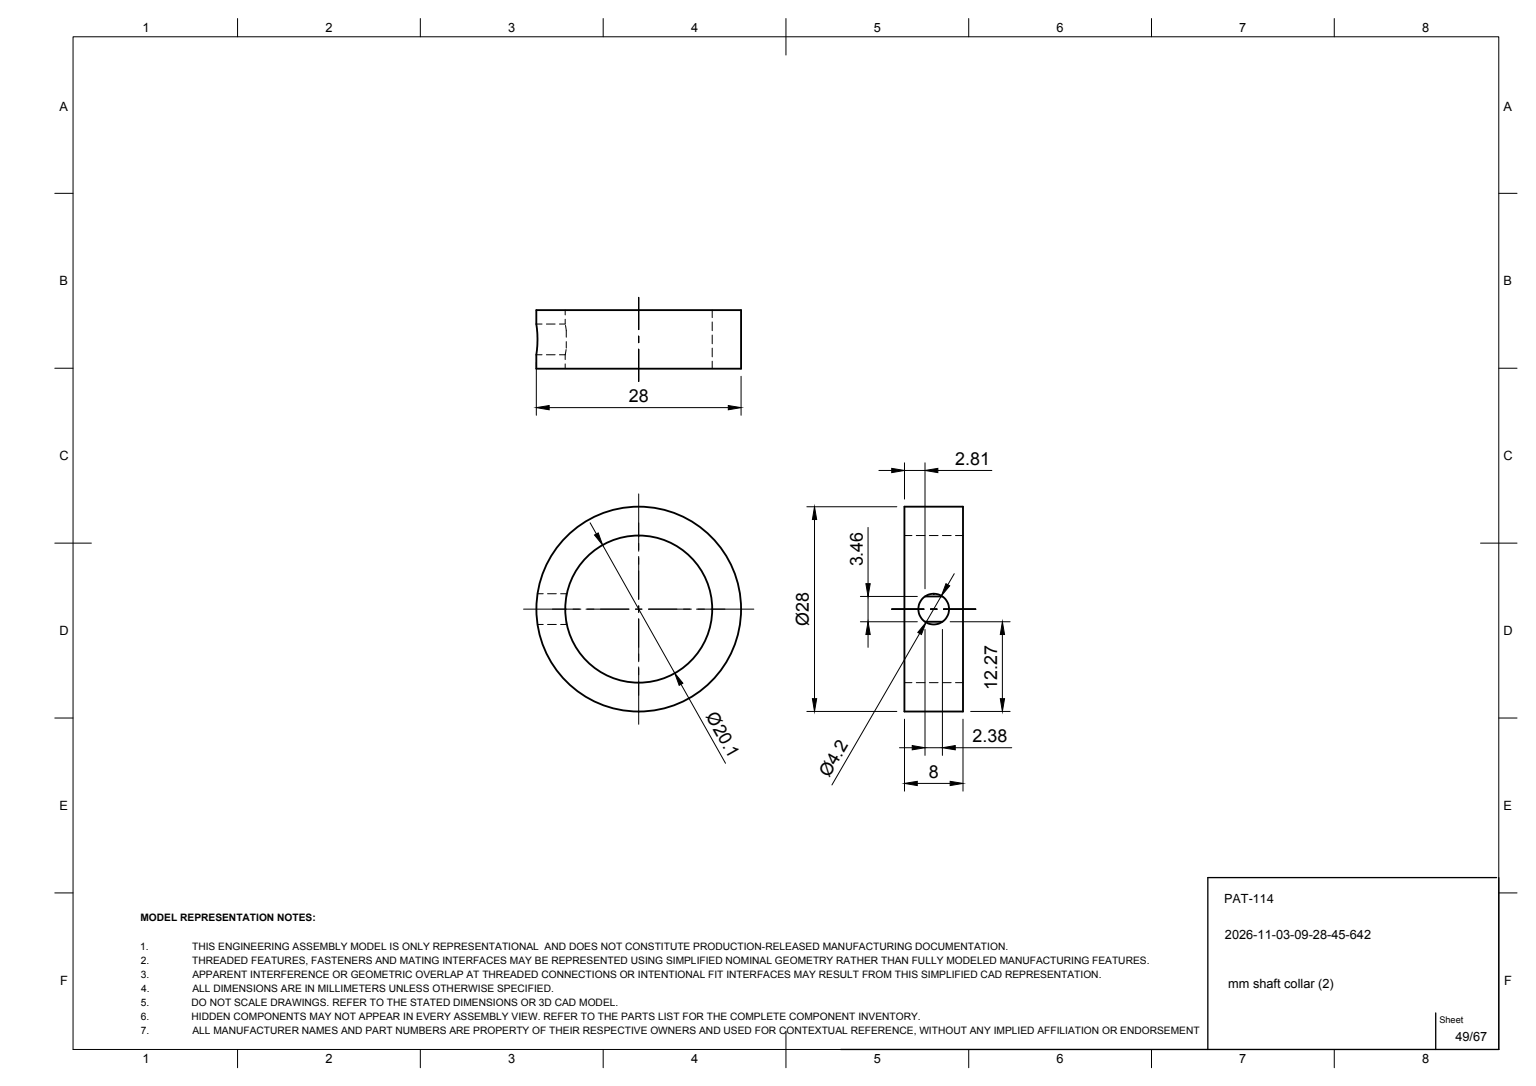
ISO-10303-21;
HEADER;
/* Generated by software containing ST-Developer
 * from STEP Tools, Inc. (www.steptools.com) 
 */

FILE_DESCRIPTION(
/* description */ ('Two-stage gear reducer in split housing'),
/* implementation_level */ '2;1');

FILE_NAME(
/* name */ 'mm shaft collar (2).step',
/* time_stamp */ '2026-10-28T03:22:31-07:00',
/* author */ (''),
/* organization */ (''),
/* preprocessor_version */ 'ST-DEVELOPER v20.2',
/* originating_system */ 'Autodesk Translation Framework v15.17.0.0',
/* authorisation */ '');

FILE_SCHEMA (('AUTOMOTIVE_DESIGN { 1 0 10303 214 3 1 1 }'));
ENDSEC;

DATA;
#10=MECHANICAL_DESIGN_GEOMETRIC_PRESENTATION_REPRESENTATION('',(#1287),#73366);
#971=B_SPLINE_CURVE_WITH_KNOTS('',3,(#37404,#37405,#37406,#37407,#37408,
#37409,#37410,#37411,#37412,#37413,#37414,#37415,#37416,#37417),
 .UNSPECIFIED.,.F.,.F.,(4,2,2,2,2,2,4),(0.756005737987032,0.793568827564648,
0.872922520054202,0.952276212543757,1.03162990503331,1.11098359752287,1.14854668710048),
 .UNSPECIFIED.);
#972=B_SPLINE_CURVE_WITH_KNOTS('',3,(#37423,#37424,#37425,#37426,#37427,
#37428,#37429,#37430,#37431,#37432,#37433,#37434,#37435,#37436,#37437,#37438,
#37439,#37440),.UNSPECIFIED.,.F.,.F.,(4,2,2,2,2,2,2,2,4),(0.,0.0792334805614376,
0.158466961122875,0.237699060165218,0.31693115920756,0.396163258249903,
0.475395357292245,0.554628837853683,0.633862318415121),.UNSPECIFIED.);
#973=B_SPLINE_CURVE_WITH_KNOTS('',3,(#37441,#37442,#37443,#37444,#37445,
#37446,#37447,#37448,#37449,#37450,#37451,#37452,#37453,#37454,#37455,#37456,
#37457,#37458),.UNSPECIFIED.,.F.,.F.,(4,2,2,2,2,2,2,2,4),(0.633862318415121,
0.713095798976558,0.792329279537995,0.871561378580338,0.950793477622681,
1.03002557666502,1.10925767570737,1.1884911562688,1.26772463683024),
 .UNSPECIFIED.);
#974=B_SPLINE_CURVE_WITH_KNOTS('',3,(#37461,#37462,#37463,#37464,#37465,
#37466,#37467,#37468,#37469,#37470,#37471,#37472,#37473,#37474),
 .UNSPECIFIED.,.F.,.F.,(4,2,2,2,2,2,4),(0.121154929624526,0.158718019202143,
0.238071711691697,0.317425404181252,0.396779096670807,0.476132789160362,
0.51369587873798),.UNSPECIFIED.);
#1160=SHAPE_REPRESENTATION_RELATIONSHIP('SRR','None',#73651,#1216);
#1216=ADVANCED_BREP_SHAPE_REPRESENTATION('',(#1356),#73347);
#1287=STYLED_ITEM('',(#73988),#1356);
#1356=MANIFOLD_SOLID_BREP('Body1',#16177);
#1560=FACE_BOUND('',#3668,.T.);
#1561=FACE_BOUND('',#3670,.T.);
#1562=FACE_BOUND('',#3672,.T.);
#1563=FACE_BOUND('',#3674,.T.);
#1870=PLANE('',#17970);
#1871=PLANE('',#17975);
#1872=PLANE('',#17982);
#1873=PLANE('',#17983);
#2565=FACE_OUTER_BOUND('',#3664,.T.);
#2566=FACE_OUTER_BOUND('',#3665,.T.);
#2567=FACE_OUTER_BOUND('',#3666,.T.);
#2568=FACE_OUTER_BOUND('',#3667,.T.);
#2569=FACE_OUTER_BOUND('',#3669,.T.);
#2570=FACE_OUTER_BOUND('',#3671,.T.);
#2571=FACE_OUTER_BOUND('',#3673,.T.);
#3664=EDGE_LOOP('',(#13043,#13044));
#3665=EDGE_LOOP('',(#13045,#13046,#13047,#13048,#13049,#13050,#13051,#13052,
#13053));
#3666=EDGE_LOOP('',(#13054,#13055,#13056));
#3667=EDGE_LOOP('',(#13057,#13058,#13059,#13060));
#3668=EDGE_LOOP('',(#13061,#13062,#13063,#13064));
#3669=EDGE_LOOP('',(#13065,#13066,#13067,#13068));
#3670=EDGE_LOOP('',(#13069,#13070));
#3671=EDGE_LOOP('',(#13071));
#3672=EDGE_LOOP('',(#13072));
#3673=EDGE_LOOP('',(#13073));
#3674=EDGE_LOOP('',(#13074));
#4684=LINE('',#37400,#5708);
#4685=LINE('',#37421,#5709);
#4686=LINE('',#37476,#5710);
#4687=LINE('',#37481,#5711);
#4688=LINE('',#37487,#5712);
#5708=VECTOR('',#21404,1.);
#5709=VECTOR('',#21411,0.21);
#5710=VECTOR('',#21416,1.);
#5711=VECTOR('',#21421,1.005);
#5712=VECTOR('',#21428,1.4);
#6624=CIRCLE('',#17971,0.21);
#6625=CIRCLE('',#17973,0.21);
#6626=CIRCLE('',#17974,0.21);
#6627=CIRCLE('',#17977,1.005);
#6628=CIRCLE('',#17978,1.005);
#6629=CIRCLE('',#17980,1.4);
#6630=CIRCLE('',#17981,1.4);
#7685=VERTEX_POINT('',#37398);
#7686=VERTEX_POINT('',#37399);
#7687=VERTEX_POINT('',#37403);
#7688=VERTEX_POINT('',#37418);
#7689=VERTEX_POINT('',#37420);
#7690=VERTEX_POINT('',#37422);
#7691=VERTEX_POINT('',#37459);
#7692=VERTEX_POINT('',#37478);
#7693=VERTEX_POINT('',#37480);
#7694=VERTEX_POINT('',#37484);
#7695=VERTEX_POINT('',#37486);
#9575=EDGE_CURVE('',#7685,#7686,#4684,.T.);
#9576=EDGE_CURVE('',#7685,#7686,#6624,.T.);
#9577=EDGE_CURVE('',#7687,#7685,#971,.T.);
#9578=EDGE_CURVE('',#7688,#7687,#6625,.T.);
#9579=EDGE_CURVE('',#7688,#7689,#4685,.T.);
#9580=EDGE_CURVE('',#7690,#7689,#972,.T.);
#9581=EDGE_CURVE('',#7689,#7690,#973,.T.);
#9582=EDGE_CURVE('',#7691,#7688,#6626,.T.);
#9583=EDGE_CURVE('',#7686,#7691,#974,.T.);
#9584=EDGE_CURVE('',#7691,#7687,#4686,.T.);
#9585=EDGE_CURVE('',#7692,#7692,#6627,.T.);
#9586=EDGE_CURVE('',#7692,#7693,#4687,.T.);
#9587=EDGE_CURVE('',#7693,#7693,#6628,.T.);
#9588=EDGE_CURVE('',#7694,#7694,#6629,.T.);
#9589=EDGE_CURVE('',#7694,#7695,#4688,.T.);
#9590=EDGE_CURVE('',#7695,#7695,#6630,.T.);
#13043=ORIENTED_EDGE('',*,*,#9575,.F.);
#13044=ORIENTED_EDGE('',*,*,#9576,.T.);
#13045=ORIENTED_EDGE('',*,*,#9577,.F.);
#13046=ORIENTED_EDGE('',*,*,#9578,.F.);
#13047=ORIENTED_EDGE('',*,*,#9579,.T.);
#13048=ORIENTED_EDGE('',*,*,#9580,.F.);
#13049=ORIENTED_EDGE('',*,*,#9581,.F.);
#13050=ORIENTED_EDGE('',*,*,#9579,.F.);
#13051=ORIENTED_EDGE('',*,*,#9582,.F.);
#13052=ORIENTED_EDGE('',*,*,#9583,.F.);
#13053=ORIENTED_EDGE('',*,*,#9576,.F.);
#13054=ORIENTED_EDGE('',*,*,#9584,.F.);
#13055=ORIENTED_EDGE('',*,*,#9582,.T.);
#13056=ORIENTED_EDGE('',*,*,#9578,.T.);
#13057=ORIENTED_EDGE('',*,*,#9585,.F.);
#13058=ORIENTED_EDGE('',*,*,#9586,.T.);
#13059=ORIENTED_EDGE('',*,*,#9587,.T.);
#13060=ORIENTED_EDGE('',*,*,#9586,.F.);
#13061=ORIENTED_EDGE('',*,*,#9583,.T.);
#13062=ORIENTED_EDGE('',*,*,#9584,.T.);
#13063=ORIENTED_EDGE('',*,*,#9577,.T.);
#13064=ORIENTED_EDGE('',*,*,#9575,.T.);
#13065=ORIENTED_EDGE('',*,*,#9588,.F.);
#13066=ORIENTED_EDGE('',*,*,#9589,.T.);
#13067=ORIENTED_EDGE('',*,*,#9590,.T.);
#13068=ORIENTED_EDGE('',*,*,#9589,.F.);
#13069=ORIENTED_EDGE('',*,*,#9580,.T.);
#13070=ORIENTED_EDGE('',*,*,#9581,.T.);
#13071=ORIENTED_EDGE('',*,*,#9588,.T.);
#13072=ORIENTED_EDGE('',*,*,#9585,.T.);
#13073=ORIENTED_EDGE('',*,*,#9590,.F.);
#13074=ORIENTED_EDGE('',*,*,#9587,.F.);
#15113=CYLINDRICAL_SURFACE('',#17972,0.21);
#15114=CYLINDRICAL_SURFACE('',#17976,1.005);
#15115=CYLINDRICAL_SURFACE('',#17979,1.4);
#15772=ADVANCED_FACE('',(#2565),#1870,.T.);
#15773=ADVANCED_FACE('',(#2566),#15113,.F.);
#15774=ADVANCED_FACE('',(#2567),#1871,.T.);
#15775=ADVANCED_FACE('',(#2568,#1560),#15114,.F.);
#15776=ADVANCED_FACE('',(#2569,#1561),#15115,.T.);
#15777=ADVANCED_FACE('',(#2570,#1562),#1872,.T.);
#15778=ADVANCED_FACE('',(#2571,#1563),#1873,.F.);
#16177=CLOSED_SHELL('',(#15772,#15773,#15774,#15775,#15776,#15777,#15778));
#17969=AXIS2_PLACEMENT_3D('',#37396,#21400,#21401);
#17970=AXIS2_PLACEMENT_3D('',#37397,#21402,#21403);
#17971=AXIS2_PLACEMENT_3D('',#37401,#21405,#21406);
#17972=AXIS2_PLACEMENT_3D('',#37402,#21407,#21408);
#17973=AXIS2_PLACEMENT_3D('',#37419,#21409,#21410);
#17974=AXIS2_PLACEMENT_3D('',#37460,#21412,#21413);
#17975=AXIS2_PLACEMENT_3D('',#37475,#21414,#21415);
#17976=AXIS2_PLACEMENT_3D('',#37477,#21417,#21418);
#17977=AXIS2_PLACEMENT_3D('',#37479,#21419,#21420);
#17978=AXIS2_PLACEMENT_3D('',#37482,#21422,#21423);
#17979=AXIS2_PLACEMENT_3D('',#37483,#21424,#21425);
#17980=AXIS2_PLACEMENT_3D('',#37485,#21426,#21427);
#17981=AXIS2_PLACEMENT_3D('',#37488,#21429,#21430);
#17982=AXIS2_PLACEMENT_3D('',#37489,#21431,#21432);
#17983=AXIS2_PLACEMENT_3D('',#37490,#21433,#21434);
#21400=DIRECTION('axis',(0.,0.,1.));
#21401=DIRECTION('refdir',(1.,0.,0.));
#21402=DIRECTION('center_axis',(0.,0.,1.));
#21403=DIRECTION('ref_axis',(1.,0.,0.));
#21404=DIRECTION('',(0.,1.,0.));
#21405=DIRECTION('center_axis',(0.,0.,1.));
#21406=DIRECTION('ref_axis',(1.,0.,0.));
#21407=DIRECTION('center_axis',(0.,0.,1.));
#21408=DIRECTION('ref_axis',(1.,0.,0.));
#21409=DIRECTION('center_axis',(0.,0.,1.));
#21410=DIRECTION('ref_axis',(1.,0.,0.));
#21411=DIRECTION('',(0.,0.,1.));
#21412=DIRECTION('center_axis',(0.,0.,1.));
#21413=DIRECTION('ref_axis',(1.,0.,0.));
#21414=DIRECTION('center_axis',(0.,0.,1.));
#21415=DIRECTION('ref_axis',(1.,0.,0.));
#21416=DIRECTION('',(0.,-1.,0.));
#21417=DIRECTION('center_axis',(0.,1.,0.));
#21418=DIRECTION('ref_axis',(1.,0.,0.));
#21419=DIRECTION('center_axis',(0.,-1.,0.));
#21420=DIRECTION('ref_axis',(1.,0.,0.));
#21421=DIRECTION('',(0.,-1.,0.));
#21422=DIRECTION('center_axis',(0.,-1.,0.));
#21423=DIRECTION('ref_axis',(1.,0.,0.));
#21424=DIRECTION('center_axis',(0.,1.,0.));
#21425=DIRECTION('ref_axis',(1.,0.,0.));
#21426=DIRECTION('center_axis',(0.,1.,0.));
#21427=DIRECTION('ref_axis',(1.,0.,0.));
#21428=DIRECTION('',(0.,-1.,0.));
#21429=DIRECTION('center_axis',(0.,1.,0.));
#21430=DIRECTION('ref_axis',(1.,0.,0.));
#21431=DIRECTION('center_axis',(0.,1.,0.));
#21432=DIRECTION('ref_axis',(1.,0.,0.));
#21433=DIRECTION('center_axis',(0.,1.,0.));
#21434=DIRECTION('ref_axis',(1.,0.,0.));
#37396=CARTESIAN_POINT('',(0.,0.,0.));
#37397=CARTESIAN_POINT('Origin',(6.,-8.2,10.99));
#37398=CARTESIAN_POINT('',(6.17298843892005,-8.31905880899792,10.99));
#37399=CARTESIAN_POINT('',(6.17298843892005,-8.08094119100208,10.99));
#37400=CARTESIAN_POINT('',(6.17298843892005,-8.6,10.99));
#37401=CARTESIAN_POINT('Origin',(6.,-8.2,10.99));
#37402=CARTESIAN_POINT('Origin',(6.,-8.2,10.99));
#37403=CARTESIAN_POINT('',(5.82701156107995,-8.31905880899792,10.99));
#37404=CARTESIAN_POINT('Ctrl Pts',(5.82701156107995,-8.31905880899792,10.99));
#37405=CARTESIAN_POINT('Ctrl Pts',(5.83440513468869,-8.3298014223953,10.9912919219764));
#37406=CARTESIAN_POINT('Ctrl Pts',(5.8427028612744,-8.33968770937275,10.992653949439));
#37407=CARTESIAN_POINT('Ctrl Pts',(5.87010792615492,-8.36709277425327,10.9967480843909));
#37408=CARTESIAN_POINT('Ctrl Pts',(5.89366983224072,-8.38324205633295,10.9996958932764));
#37409=CARTESIAN_POINT('Ctrl Pts',(5.94538709536759,-8.40469779396491,11.0038502947236));
#37410=CARTESIAN_POINT('Ctrl Pts',(5.97354876917015,-8.41,11.005));
#37411=CARTESIAN_POINT('Ctrl Pts',(6.02645123082985,-8.41,11.005));
#37412=CARTESIAN_POINT('Ctrl Pts',(6.05461290463241,-8.40469779396491,11.0038502947236));
#37413=CARTESIAN_POINT('Ctrl Pts',(6.10633016775928,-8.38324205633295,10.9996958932764));
#37414=CARTESIAN_POINT('Ctrl Pts',(6.12989207384508,-8.36709277425327,10.9967480843909));
#37415=CARTESIAN_POINT('Ctrl Pts',(6.1572971387256,-8.33968770937275,10.992653949439));
#37416=CARTESIAN_POINT('Ctrl Pts',(6.16559486531131,-8.3298014223953,10.9912919219764));
#37417=CARTESIAN_POINT('Ctrl Pts',(6.17298843892005,-8.31905880899792,10.99));
#37418=CARTESIAN_POINT('',(5.79,-8.2,10.99));
#37419=CARTESIAN_POINT('Origin',(6.,-8.2,10.99));
#37420=CARTESIAN_POINT('',(5.79,-8.2,11.38416039533));
#37421=CARTESIAN_POINT('',(5.79,-8.2,10.99));
#37422=CARTESIAN_POINT('',(6.21,-8.2,11.38416039533));
#37423=CARTESIAN_POINT('Ctrl Pts',(6.21,-8.2,11.38416039533));
#37424=CARTESIAN_POINT('Ctrl Pts',(6.21,-8.22641116018714,11.38416039533));
#37425=CARTESIAN_POINT('Ctrl Pts',(6.20471354911189,-8.2545550596171,11.3849944296993));
#37426=CARTESIAN_POINT('Ctrl Pts',(6.18326999585849,-8.30628264999174,11.3879947099895));
#37427=CARTESIAN_POINT('Ctrl Pts',(6.16711503760643,-8.32986981049192,11.3901162943626));
#37428=CARTESIAN_POINT('Ctrl Pts',(6.12987013519678,-8.36711471290156,11.394089123191));
#37429=CARTESIAN_POINT('Ctrl Pts',(6.10628283459019,-8.38326992585508,11.3962002442067));
#37430=CARTESIAN_POINT('Ctrl Pts',(6.05455476560391,-8.40471366447292,11.3991765222353));
#37431=CARTESIAN_POINT('Ctrl Pts',(6.02641069968078,-8.41,11.4));
#37432=CARTESIAN_POINT('Ctrl Pts',(5.97358930031922,-8.41,11.4));
#37433=CARTESIAN_POINT('Ctrl Pts',(5.94544523439609,-8.40471366447292,11.3991765222353));
#37434=CARTESIAN_POINT('Ctrl Pts',(5.89371716540981,-8.38326992585508,11.3962002442067));
#37435=CARTESIAN_POINT('Ctrl Pts',(5.87012986480322,-8.36711471290156,11.394089123191));
#37436=CARTESIAN_POINT('Ctrl Pts',(5.83288496239357,-8.32986981049192,11.3901162943626));
#37437=CARTESIAN_POINT('Ctrl Pts',(5.81673000414151,-8.30628264999174,11.3879947099895));
#37438=CARTESIAN_POINT('Ctrl Pts',(5.79528645088811,-8.2545550596171,11.3849944296993));
#37439=CARTESIAN_POINT('Ctrl Pts',(5.79,-8.22641116018714,11.38416039533));
#37440=CARTESIAN_POINT('Ctrl Pts',(5.79,-8.2,11.38416039533));
#37441=CARTESIAN_POINT('Ctrl Pts',(5.79,-8.2,11.38416039533));
#37442=CARTESIAN_POINT('Ctrl Pts',(5.79,-8.17358883981285,11.38416039533));
#37443=CARTESIAN_POINT('Ctrl Pts',(5.79528645088811,-8.1454449403829,11.3849944296993));
#37444=CARTESIAN_POINT('Ctrl Pts',(5.81673000414151,-8.09371735000826,11.3879947099895));
#37445=CARTESIAN_POINT('Ctrl Pts',(5.83288496239357,-8.07013018950807,11.3901162943626));
#37446=CARTESIAN_POINT('Ctrl Pts',(5.87012986480322,-8.03288528709843,11.394089123191));
#37447=CARTESIAN_POINT('Ctrl Pts',(5.89371716540981,-8.01673007414492,11.3962002442067));
#37448=CARTESIAN_POINT('Ctrl Pts',(5.94544523439609,-7.99528633552708,11.3991765222353));
#37449=CARTESIAN_POINT('Ctrl Pts',(5.97358930031922,-7.99,11.4));
#37450=CARTESIAN_POINT('Ctrl Pts',(6.02641069968078,-7.99,11.4));
#37451=CARTESIAN_POINT('Ctrl Pts',(6.05455476560391,-7.99528633552708,11.3991765222353));
#37452=CARTESIAN_POINT('Ctrl Pts',(6.10628283459019,-8.01673007414492,11.3962002442067));
#37453=CARTESIAN_POINT('Ctrl Pts',(6.12987013519678,-8.03288528709843,11.394089123191));
#37454=CARTESIAN_POINT('Ctrl Pts',(6.16711503760642,-8.07013018950807,11.3901162943626));
#37455=CARTESIAN_POINT('Ctrl Pts',(6.18326999585848,-8.09371735000826,11.3879947099895));
#37456=CARTESIAN_POINT('Ctrl Pts',(6.20471354911189,-8.1454449403829,11.3849944296993));
#37457=CARTESIAN_POINT('Ctrl Pts',(6.21,-8.17358883981285,11.38416039533));
#37458=CARTESIAN_POINT('Ctrl Pts',(6.21,-8.2,11.38416039533));
#37459=CARTESIAN_POINT('',(5.82701156107995,-8.08094119100208,10.99));
#37460=CARTESIAN_POINT('Origin',(6.,-8.2,10.99));
#37461=CARTESIAN_POINT('Ctrl Pts',(6.17298843892005,-8.08094119100207,10.99));
#37462=CARTESIAN_POINT('Ctrl Pts',(6.16559486531131,-8.0701985776047,10.9912919219764));
#37463=CARTESIAN_POINT('Ctrl Pts',(6.1572971387256,-8.06031229062725,10.992653949439));
#37464=CARTESIAN_POINT('Ctrl Pts',(6.12989207384508,-8.03290722574673,10.9967480843909));
#37465=CARTESIAN_POINT('Ctrl Pts',(6.10633016775929,-8.01675794366705,10.9996958932764));
#37466=CARTESIAN_POINT('Ctrl Pts',(6.05461290463241,-7.99530220603509,11.0038502947236));
#37467=CARTESIAN_POINT('Ctrl Pts',(6.02645123082985,-7.99,11.005));
#37468=CARTESIAN_POINT('Ctrl Pts',(5.97354876917015,-7.99,11.005));
#37469=CARTESIAN_POINT('Ctrl Pts',(5.94538709536759,-7.99530220603509,11.0038502947236));
#37470=CARTESIAN_POINT('Ctrl Pts',(5.89366983224071,-8.01675794366705,10.9996958932764));
#37471=CARTESIAN_POINT('Ctrl Pts',(5.87010792615492,-8.03290722574673,10.9967480843909));
#37472=CARTESIAN_POINT('Ctrl Pts',(5.8427028612744,-8.06031229062725,10.992653949439));
#37473=CARTESIAN_POINT('Ctrl Pts',(5.83440513468869,-8.0701985776047,10.9912919219764));
#37474=CARTESIAN_POINT('Ctrl Pts',(5.82701156107995,-8.08094119100208,10.99));
#37475=CARTESIAN_POINT('Origin',(6.,-8.2,10.99));
#37476=CARTESIAN_POINT('',(5.82701156107995,-8.6,10.99));
#37477=CARTESIAN_POINT('Origin',(6.,-8.6,10.));
#37478=CARTESIAN_POINT('',(4.995,-7.8,10.));
#37479=CARTESIAN_POINT('Origin',(6.,-7.8,10.));
#37480=CARTESIAN_POINT('',(4.995,-8.6,10.));
#37481=CARTESIAN_POINT('',(4.995,-8.6,10.));
#37482=CARTESIAN_POINT('Origin',(6.,-8.6,10.));
#37483=CARTESIAN_POINT('Origin',(6.,-8.6,10.));
#37484=CARTESIAN_POINT('',(4.6,-7.8,10.));
#37485=CARTESIAN_POINT('Origin',(6.,-7.8,10.));
#37486=CARTESIAN_POINT('',(4.6,-8.6,10.));
#37487=CARTESIAN_POINT('',(4.6,-8.6,10.));
#37488=CARTESIAN_POINT('Origin',(6.,-8.6,10.));
#37489=CARTESIAN_POINT('Origin',(6.,-7.8,10.));
#37490=CARTESIAN_POINT('Origin',(6.,-8.6,10.));
#73283=UNCERTAINTY_MEASURE_WITH_UNIT(LENGTH_MEASURE(0.001),#73367,
'DISTANCE_ACCURACY_VALUE',
'Maximum model space distance between geometric entities at asserted c
onnectivities');
#73302=UNCERTAINTY_MEASURE_WITH_UNIT(LENGTH_MEASURE(0.001),#73367,
'DISTANCE_ACCURACY_VALUE',
'Maximum model space distance between geometric entities at asserted c
onnectivities');
#73347=(
GEOMETRIC_REPRESENTATION_CONTEXT(3)
GLOBAL_UNCERTAINTY_ASSIGNED_CONTEXT((#73283))
GLOBAL_UNIT_ASSIGNED_CONTEXT((#73367,#73369,#73370))
REPRESENTATION_CONTEXT('','3D')
);
#73366=(
GEOMETRIC_REPRESENTATION_CONTEXT(3)
GLOBAL_UNCERTAINTY_ASSIGNED_CONTEXT((#73302))
GLOBAL_UNIT_ASSIGNED_CONTEXT((#73367,#73369,#73370))
REPRESENTATION_CONTEXT('','3D')
);
#73367=(
LENGTH_UNIT()
NAMED_UNIT(*)
SI_UNIT(.CENTI.,.METRE.)
);
#73369=(
NAMED_UNIT(*)
PLANE_ANGLE_UNIT()
SI_UNIT($,.RADIAN.)
);
#73370=(
NAMED_UNIT(*)
SI_UNIT($,.STERADIAN.)
SOLID_ANGLE_UNIT()
);
#73415=SHAPE_DEFINITION_REPRESENTATION(#73548,#73651);
#73548=PRODUCT_DEFINITION_SHAPE('',$,#73715);
#73651=SHAPE_REPRESENTATION('',(#17969),#73347);
#73670=PRODUCT_DEFINITION_CONTEXT('part definition',#73861,'design');
#73715=PRODUCT_DEFINITION('mm shaft collar (2)','mm shaft collar (2)',#73778,
#73670);
#73778=PRODUCT_DEFINITION_FORMATION('',$,#73907);
#73861=APPLICATION_CONTEXT(
'Core Data for Automotive Mechanical Design Process');
#73862=PRODUCT_CONTEXT('part definition',#73861,'mechanical');
#73907=PRODUCT('mm shaft collar (2)','mm shaft collar (2)',
'mm shaft collar (2)',(#73862));
#73982=COLOUR_RGB('Grey',0.48,0.52,0.57);
#73983=FILL_AREA_STYLE_COLOUR('',#73982);
#73984=FILL_AREA_STYLE('',(#73983));
#73985=SURFACE_STYLE_FILL_AREA(#73984);
#73986=SURFACE_SIDE_STYLE('',(#73985));
#73987=SURFACE_STYLE_USAGE(.BOTH.,#73986);
#73988=PRESENTATION_STYLE_ASSIGNMENT((#73987));
ENDSEC;
END-ISO-10303-21;
